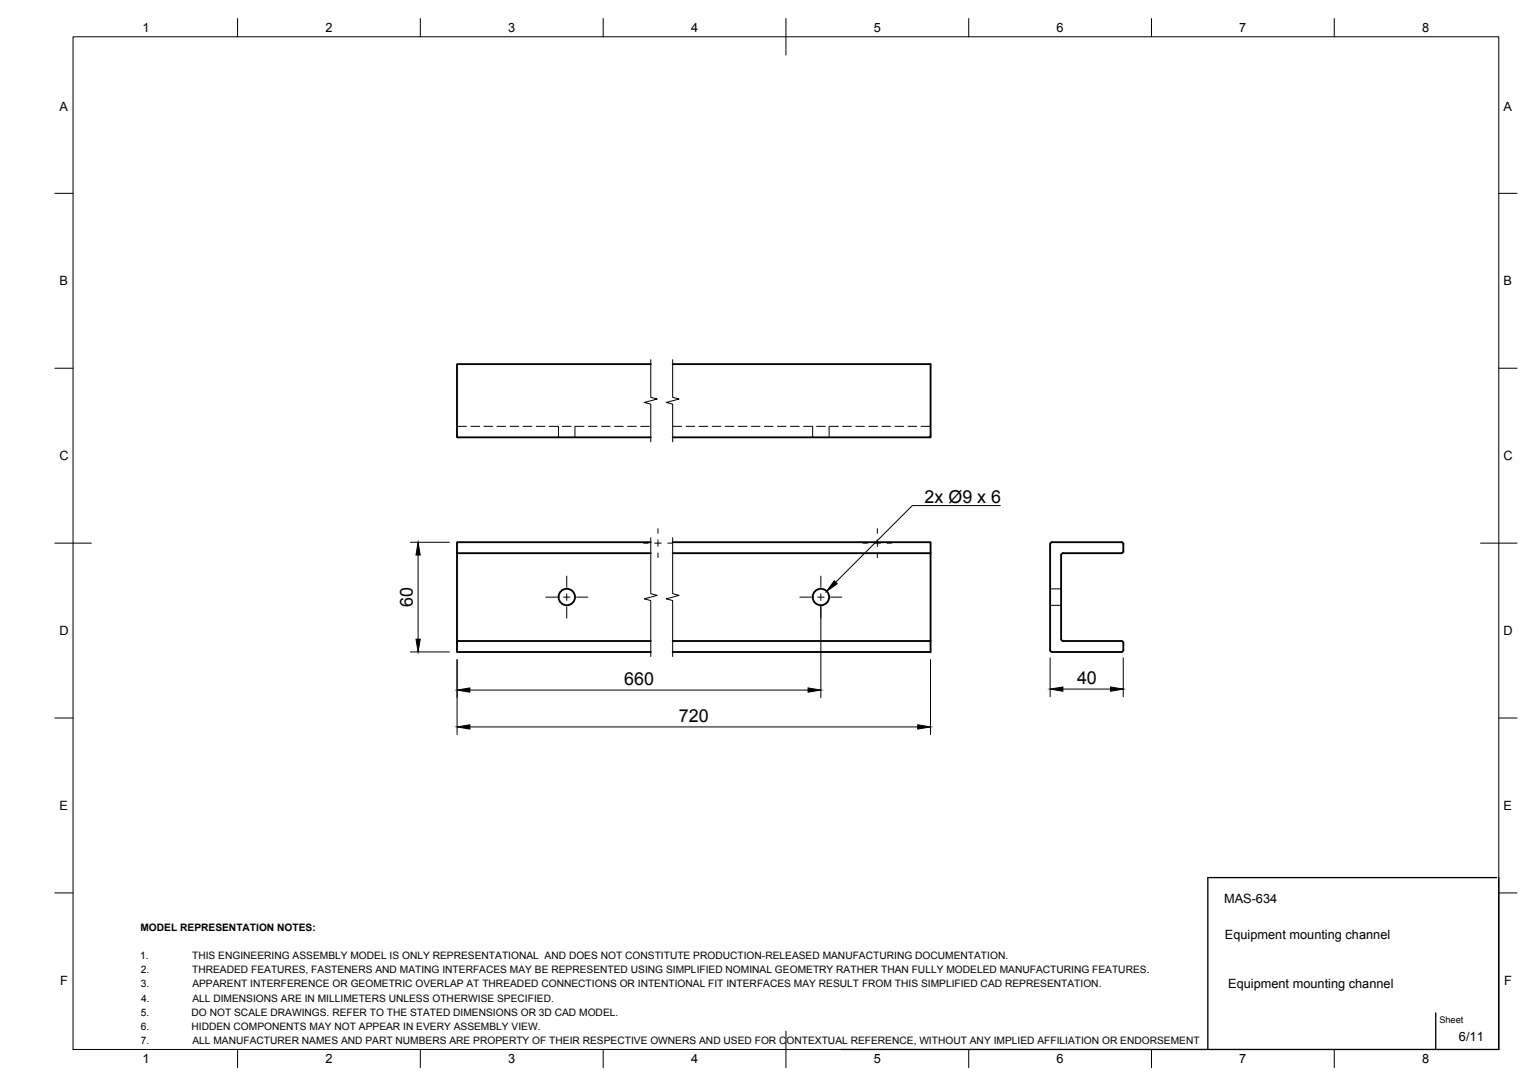
ISO-10303-21;
HEADER;
/* Generated by software containing ST-Developer
 * from STEP Tools, Inc. (www.steptools.com) 
 */

FILE_DESCRIPTION(
/* description */ ('Independent AHU equipment rack. Nominal800x600 frame on1000long40squa
re aluminum posts; two removable notched shelves; welded perimeter/cro
ss rails and rear gussets; two mounting channels; four isolation pads 
and anchor-ready feet. Imported native extrusion library retained and 
cut-length parameters customized per family. Shelf hardware uses model
ed M6 rivet nuts and screws. Weld design, floor anchors and load ratin
g require engineering selection.'),
/* implementation_level */ '2;1');

FILE_NAME(
/* name */ 'Equipment mounting channel.step',
/* time_stamp */ '2026-11-07T19:04:45-08:00',
/* author */ (''),
/* organization */ (''),
/* preprocessor_version */ 'ST-DEVELOPER v20.2',
/* originating_system */ 'Autodesk Translation Framework v15.17.0.0',
/* authorisation */ '');

FILE_SCHEMA (('AUTOMOTIVE_DESIGN { 1 0 10303 214 3 1 1 }'));
ENDSEC;

DATA;
#10=MECHANICAL_DESIGN_GEOMETRIC_PRESENTATION_REPRESENTATION('',(#338),#9777);
#316=SHAPE_REPRESENTATION_RELATIONSHIP('SRR','None',#9860,#327);
#327=ADVANCED_BREP_SHAPE_REPRESENTATION('',(#349),#9769);
#338=STYLED_ITEM('',(#9923),#349);
#349=MANIFOLD_SOLID_BREP('Aluminum channel profile',#3843);
#367=FACE_BOUND('',#771,.T.);
#368=FACE_BOUND('',#772,.T.);
#369=FACE_BOUND('',#779,.T.);
#370=FACE_BOUND('',#780,.T.);
#440=PLANE('',#4095);
#441=PLANE('',#4103);
#442=PLANE('',#4108);
#443=PLANE('',#4113);
#444=PLANE('',#4116);
#445=PLANE('',#4121);
#446=PLANE('',#4122);
#447=PLANE('',#4123);
#448=PLANE('',#4124);
#449=PLANE('',#4125);
#558=FACE_OUTER_BOUND('',#766,.T.);
#559=FACE_OUTER_BOUND('',#767,.T.);
#560=FACE_OUTER_BOUND('',#768,.T.);
#561=FACE_OUTER_BOUND('',#769,.T.);
#562=FACE_OUTER_BOUND('',#770,.T.);
#563=FACE_OUTER_BOUND('',#773,.T.);
#564=FACE_OUTER_BOUND('',#774,.T.);
#565=FACE_OUTER_BOUND('',#775,.T.);
#566=FACE_OUTER_BOUND('',#776,.T.);
#567=FACE_OUTER_BOUND('',#777,.T.);
#568=FACE_OUTER_BOUND('',#778,.T.);
#569=FACE_OUTER_BOUND('',#781,.T.);
#570=FACE_OUTER_BOUND('',#782,.T.);
#571=FACE_OUTER_BOUND('',#783,.T.);
#572=FACE_OUTER_BOUND('',#784,.T.);
#573=FACE_OUTER_BOUND('',#785,.T.);
#574=FACE_OUTER_BOUND('',#786,.T.);
#575=FACE_OUTER_BOUND('',#787,.T.);
#576=FACE_OUTER_BOUND('',#788,.T.);
#577=FACE_OUTER_BOUND('',#789,.T.);
#766=EDGE_LOOP('',(#2815,#2816,#2817,#2818));
#767=EDGE_LOOP('',(#2819,#2820,#2821,#2822));
#768=EDGE_LOOP('',(#2823,#2824,#2825,#2826));
#769=EDGE_LOOP('',(#2827,#2828,#2829,#2830,#2831,#2832,#2833,#2834,#2835,
#2836,#2837,#2838,#2839,#2840,#2841,#2842));
#770=EDGE_LOOP('',(#2843,#2844,#2845,#2846));
#771=EDGE_LOOP('',(#2847));
#772=EDGE_LOOP('',(#2848));
#773=EDGE_LOOP('',(#2849,#2850,#2851,#2852));
#774=EDGE_LOOP('',(#2853,#2854,#2855,#2856));
#775=EDGE_LOOP('',(#2857,#2858,#2859,#2860));
#776=EDGE_LOOP('',(#2861,#2862,#2863,#2864));
#777=EDGE_LOOP('',(#2865,#2866,#2867,#2868));
#778=EDGE_LOOP('',(#2869,#2870,#2871,#2872));
#779=EDGE_LOOP('',(#2873));
#780=EDGE_LOOP('',(#2874));
#781=EDGE_LOOP('',(#2875,#2876,#2877,#2878));
#782=EDGE_LOOP('',(#2879,#2880,#2881,#2882));
#783=EDGE_LOOP('',(#2883,#2884,#2885,#2886));
#784=EDGE_LOOP('',(#2887,#2888,#2889,#2890));
#785=EDGE_LOOP('',(#2891,#2892,#2893,#2894));
#786=EDGE_LOOP('',(#2895,#2896,#2897,#2898));
#787=EDGE_LOOP('',(#2899,#2900,#2901,#2902));
#788=EDGE_LOOP('',(#2903,#2904,#2905,#2906));
#789=EDGE_LOOP('',(#2907,#2908,#2909,#2910,#2911,#2912,#2913,#2914,#2915,
#2916,#2917,#2918,#2919,#2920,#2921,#2922));
#1049=LINE('',#5718,#1342);
#1050=LINE('',#5724,#1343);
#1051=LINE('',#5731,#1344);
#1052=LINE('',#5734,#1345);
#1053=LINE('',#5737,#1346);
#1054=LINE('',#5741,#1347);
#1055=LINE('',#5745,#1348);
#1056=LINE('',#5749,#1349);
#1057=LINE('',#5753,#1350);
#1058=LINE('',#5757,#1351);
#1059=LINE('',#5761,#1352);
#1060=LINE('',#5764,#1353);
#1061=LINE('',#5767,#1354);
#1062=LINE('',#5768,#1355);
#1063=LINE('',#5772,#1356);
#1064=LINE('',#5775,#1357);
#1065=LINE('',#5778,#1358);
#1066=LINE('',#5781,#1359);
#1067=LINE('',#5782,#1360);
#1068=LINE('',#5786,#1361);
#1069=LINE('',#5791,#1362);
#1070=LINE('',#5792,#1363);
#1071=LINE('',#5795,#1364);
#1072=LINE('',#5796,#1365);
#1073=LINE('',#5800,#1366);
#1074=LINE('',#5803,#1367);
#1075=LINE('',#5804,#1368);
#1076=LINE('',#5808,#1369);
#1077=LINE('',#5811,#1370);
#1078=LINE('',#5814,#1371);
#1079=LINE('',#5816,#1372);
#1080=LINE('',#5818,#1373);
#1081=LINE('',#5820,#1374);
#1082=LINE('',#5822,#1375);
#1342=VECTOR('',#4680,4.5);
#1343=VECTOR('',#4687,4.5);
#1344=VECTOR('',#4694,10.);
#1345=VECTOR('',#4697,10.);
#1346=VECTOR('',#4700,10.);
#1347=VECTOR('',#4703,10.);
#1348=VECTOR('',#4706,10.);
#1349=VECTOR('',#4709,10.);
#1350=VECTOR('',#4712,10.);
#1351=VECTOR('',#4715,10.);
#1352=VECTOR('',#4718,10.);
#1353=VECTOR('',#4721,10.);
#1354=VECTOR('',#4724,10.);
#1355=VECTOR('',#4725,10.);
#1356=VECTOR('',#4730,10.);
#1357=VECTOR('',#4733,10.);
#1358=VECTOR('',#4736,10.);
#1359=VECTOR('',#4739,10.);
#1360=VECTOR('',#4740,10.);
#1361=VECTOR('',#4745,10.);
#1362=VECTOR('',#4750,10.);
#1363=VECTOR('',#4751,10.);
#1364=VECTOR('',#4754,10.);
#1365=VECTOR('',#4755,10.);
#1366=VECTOR('',#4760,10.);
#1367=VECTOR('',#4763,10.);
#1368=VECTOR('',#4764,10.);
#1369=VECTOR('',#4769,10.);
#1370=VECTOR('',#4772,10.);
#1371=VECTOR('',#4775,10.);
#1372=VECTOR('',#4778,10.);
#1373=VECTOR('',#4781,10.);
#1374=VECTOR('',#4784,10.);
#1375=VECTOR('',#4787,10.);
#1589=CIRCLE('',#4087,4.5);
#1590=CIRCLE('',#4088,4.5);
#1591=CIRCLE('',#4090,4.5);
#1592=CIRCLE('',#4091,4.5);
#1593=CIRCLE('',#4093,1.);
#1594=CIRCLE('',#4094,1.);
#1595=CIRCLE('',#4096,1.);
#1596=CIRCLE('',#4097,1.);
#1597=CIRCLE('',#4098,1.);
#1598=CIRCLE('',#4099,1.);
#1599=CIRCLE('',#4100,1.);
#1600=CIRCLE('',#4101,1.);
#1601=CIRCLE('',#4102,1.);
#1602=CIRCLE('',#4105,1.);
#1603=CIRCLE('',#4107,1.);
#1604=CIRCLE('',#4110,1.);
#1605=CIRCLE('',#4112,1.);
#1606=CIRCLE('',#4115,1.);
#1607=CIRCLE('',#4118,1.);
#1608=CIRCLE('',#4120,1.);
#1760=VERTEX_POINT('',#5715);
#1761=VERTEX_POINT('',#5717);
#1762=VERTEX_POINT('',#5721);
#1763=VERTEX_POINT('',#5723);
#1764=VERTEX_POINT('',#5727);
#1765=VERTEX_POINT('',#5728);
#1766=VERTEX_POINT('',#5730);
#1767=VERTEX_POINT('',#5732);
#1768=VERTEX_POINT('',#5736);
#1769=VERTEX_POINT('',#5738);
#1770=VERTEX_POINT('',#5740);
#1771=VERTEX_POINT('',#5742);
#1772=VERTEX_POINT('',#5744);
#1773=VERTEX_POINT('',#5746);
#1774=VERTEX_POINT('',#5748);
#1775=VERTEX_POINT('',#5750);
#1776=VERTEX_POINT('',#5752);
#1777=VERTEX_POINT('',#5754);
#1778=VERTEX_POINT('',#5756);
#1779=VERTEX_POINT('',#5758);
#1780=VERTEX_POINT('',#5760);
#1781=VERTEX_POINT('',#5762);
#1782=VERTEX_POINT('',#5766);
#1783=VERTEX_POINT('',#5770);
#1784=VERTEX_POINT('',#5774);
#1785=VERTEX_POINT('',#5776);
#1786=VERTEX_POINT('',#5780);
#1787=VERTEX_POINT('',#5784);
#1788=VERTEX_POINT('',#5788);
#1789=VERTEX_POINT('',#5789);
#1790=VERTEX_POINT('',#5794);
#1791=VERTEX_POINT('',#5798);
#1792=VERTEX_POINT('',#5802);
#1793=VERTEX_POINT('',#5806);
#1794=VERTEX_POINT('',#5810);
#1795=VERTEX_POINT('',#5812);
#2152=EDGE_CURVE('',#1760,#1760,#1589,.T.);
#2153=EDGE_CURVE('',#1760,#1761,#1049,.T.);
#2154=EDGE_CURVE('',#1761,#1761,#1590,.T.);
#2155=EDGE_CURVE('',#1762,#1762,#1591,.T.);
#2156=EDGE_CURVE('',#1762,#1763,#1050,.T.);
#2157=EDGE_CURVE('',#1763,#1763,#1592,.T.);
#2158=EDGE_CURVE('',#1764,#1765,#1593,.T.);
#2159=EDGE_CURVE('',#1765,#1766,#1051,.T.);
#2160=EDGE_CURVE('',#1766,#1767,#1594,.T.);
#2161=EDGE_CURVE('',#1767,#1764,#1052,.T.);
#2162=EDGE_CURVE('',#1764,#1768,#1053,.T.);
#2163=EDGE_CURVE('',#1769,#1768,#1595,.T.);
#2164=EDGE_CURVE('',#1769,#1770,#1054,.T.);
#2165=EDGE_CURVE('',#1771,#1770,#1596,.T.);
#2166=EDGE_CURVE('',#1771,#1772,#1055,.T.);
#2167=EDGE_CURVE('',#1773,#1772,#1597,.T.);
#2168=EDGE_CURVE('',#1773,#1774,#1056,.T.);
#2169=EDGE_CURVE('',#1775,#1774,#1598,.T.);
#2170=EDGE_CURVE('',#1775,#1776,#1057,.T.);
#2171=EDGE_CURVE('',#1777,#1776,#1599,.T.);
#2172=EDGE_CURVE('',#1777,#1778,#1058,.T.);
#2173=EDGE_CURVE('',#1779,#1778,#1600,.T.);
#2174=EDGE_CURVE('',#1779,#1780,#1059,.T.);
#2175=EDGE_CURVE('',#1781,#1780,#1601,.T.);
#2176=EDGE_CURVE('',#1781,#1765,#1060,.T.);
#2177=EDGE_CURVE('',#1767,#1782,#1061,.T.);
#2178=EDGE_CURVE('',#1768,#1782,#1062,.T.);
#2179=EDGE_CURVE('',#1782,#1783,#1602,.T.);
#2180=EDGE_CURVE('',#1783,#1769,#1063,.T.);
#2181=EDGE_CURVE('',#1770,#1784,#1064,.T.);
#2182=EDGE_CURVE('',#1784,#1785,#1603,.T.);
#2183=EDGE_CURVE('',#1785,#1771,#1065,.T.);
#2184=EDGE_CURVE('',#1785,#1786,#1066,.T.);
#2185=EDGE_CURVE('',#1772,#1786,#1067,.T.);
#2186=EDGE_CURVE('',#1786,#1787,#1604,.T.);
#2187=EDGE_CURVE('',#1787,#1773,#1068,.T.);
#2188=EDGE_CURVE('',#1788,#1789,#1605,.T.);
#2189=EDGE_CURVE('',#1789,#1775,#1069,.T.);
#2190=EDGE_CURVE('',#1774,#1788,#1070,.T.);
#2191=EDGE_CURVE('',#1789,#1790,#1071,.T.);
#2192=EDGE_CURVE('',#1776,#1790,#1072,.T.);
#2193=EDGE_CURVE('',#1790,#1791,#1606,.T.);
#2194=EDGE_CURVE('',#1791,#1777,#1073,.T.);
#2195=EDGE_CURVE('',#1791,#1792,#1074,.T.);
#2196=EDGE_CURVE('',#1778,#1792,#1075,.T.);
#2197=EDGE_CURVE('',#1792,#1793,#1607,.T.);
#2198=EDGE_CURVE('',#1793,#1779,#1076,.T.);
#2199=EDGE_CURVE('',#1780,#1794,#1077,.T.);
#2200=EDGE_CURVE('',#1794,#1795,#1608,.T.);
#2201=EDGE_CURVE('',#1795,#1781,#1078,.T.);
#2202=EDGE_CURVE('',#1795,#1766,#1079,.T.);
#2203=EDGE_CURVE('',#1793,#1794,#1080,.T.);
#2204=EDGE_CURVE('',#1787,#1788,#1081,.T.);
#2205=EDGE_CURVE('',#1783,#1784,#1082,.T.);
#2815=ORIENTED_EDGE('',*,*,#2152,.F.);
#2816=ORIENTED_EDGE('',*,*,#2153,.T.);
#2817=ORIENTED_EDGE('',*,*,#2154,.F.);
#2818=ORIENTED_EDGE('',*,*,#2153,.F.);
#2819=ORIENTED_EDGE('',*,*,#2155,.F.);
#2820=ORIENTED_EDGE('',*,*,#2156,.T.);
#2821=ORIENTED_EDGE('',*,*,#2157,.F.);
#2822=ORIENTED_EDGE('',*,*,#2156,.F.);
#2823=ORIENTED_EDGE('',*,*,#2158,.T.);
#2824=ORIENTED_EDGE('',*,*,#2159,.T.);
#2825=ORIENTED_EDGE('',*,*,#2160,.T.);
#2826=ORIENTED_EDGE('',*,*,#2161,.T.);
#2827=ORIENTED_EDGE('',*,*,#2158,.F.);
#2828=ORIENTED_EDGE('',*,*,#2162,.T.);
#2829=ORIENTED_EDGE('',*,*,#2163,.F.);
#2830=ORIENTED_EDGE('',*,*,#2164,.T.);
#2831=ORIENTED_EDGE('',*,*,#2165,.F.);
#2832=ORIENTED_EDGE('',*,*,#2166,.T.);
#2833=ORIENTED_EDGE('',*,*,#2167,.F.);
#2834=ORIENTED_EDGE('',*,*,#2168,.T.);
#2835=ORIENTED_EDGE('',*,*,#2169,.F.);
#2836=ORIENTED_EDGE('',*,*,#2170,.T.);
#2837=ORIENTED_EDGE('',*,*,#2171,.F.);
#2838=ORIENTED_EDGE('',*,*,#2172,.T.);
#2839=ORIENTED_EDGE('',*,*,#2173,.F.);
#2840=ORIENTED_EDGE('',*,*,#2174,.T.);
#2841=ORIENTED_EDGE('',*,*,#2175,.F.);
#2842=ORIENTED_EDGE('',*,*,#2176,.T.);
#2843=ORIENTED_EDGE('',*,*,#2161,.F.);
#2844=ORIENTED_EDGE('',*,*,#2177,.T.);
#2845=ORIENTED_EDGE('',*,*,#2178,.F.);
#2846=ORIENTED_EDGE('',*,*,#2162,.F.);
#2847=ORIENTED_EDGE('',*,*,#2154,.T.);
#2848=ORIENTED_EDGE('',*,*,#2157,.T.);
#2849=ORIENTED_EDGE('',*,*,#2163,.T.);
#2850=ORIENTED_EDGE('',*,*,#2178,.T.);
#2851=ORIENTED_EDGE('',*,*,#2179,.T.);
#2852=ORIENTED_EDGE('',*,*,#2180,.T.);
#2853=ORIENTED_EDGE('',*,*,#2165,.T.);
#2854=ORIENTED_EDGE('',*,*,#2181,.T.);
#2855=ORIENTED_EDGE('',*,*,#2182,.T.);
#2856=ORIENTED_EDGE('',*,*,#2183,.T.);
#2857=ORIENTED_EDGE('',*,*,#2183,.F.);
#2858=ORIENTED_EDGE('',*,*,#2184,.T.);
#2859=ORIENTED_EDGE('',*,*,#2185,.F.);
#2860=ORIENTED_EDGE('',*,*,#2166,.F.);
#2861=ORIENTED_EDGE('',*,*,#2167,.T.);
#2862=ORIENTED_EDGE('',*,*,#2185,.T.);
#2863=ORIENTED_EDGE('',*,*,#2186,.T.);
#2864=ORIENTED_EDGE('',*,*,#2187,.T.);
#2865=ORIENTED_EDGE('',*,*,#2188,.T.);
#2866=ORIENTED_EDGE('',*,*,#2189,.T.);
#2867=ORIENTED_EDGE('',*,*,#2169,.T.);
#2868=ORIENTED_EDGE('',*,*,#2190,.T.);
#2869=ORIENTED_EDGE('',*,*,#2189,.F.);
#2870=ORIENTED_EDGE('',*,*,#2191,.T.);
#2871=ORIENTED_EDGE('',*,*,#2192,.F.);
#2872=ORIENTED_EDGE('',*,*,#2170,.F.);
#2873=ORIENTED_EDGE('',*,*,#2152,.T.);
#2874=ORIENTED_EDGE('',*,*,#2155,.T.);
#2875=ORIENTED_EDGE('',*,*,#2193,.T.);
#2876=ORIENTED_EDGE('',*,*,#2194,.T.);
#2877=ORIENTED_EDGE('',*,*,#2171,.T.);
#2878=ORIENTED_EDGE('',*,*,#2192,.T.);
#2879=ORIENTED_EDGE('',*,*,#2194,.F.);
#2880=ORIENTED_EDGE('',*,*,#2195,.T.);
#2881=ORIENTED_EDGE('',*,*,#2196,.F.);
#2882=ORIENTED_EDGE('',*,*,#2172,.F.);
#2883=ORIENTED_EDGE('',*,*,#2173,.T.);
#2884=ORIENTED_EDGE('',*,*,#2196,.T.);
#2885=ORIENTED_EDGE('',*,*,#2197,.T.);
#2886=ORIENTED_EDGE('',*,*,#2198,.T.);
#2887=ORIENTED_EDGE('',*,*,#2175,.T.);
#2888=ORIENTED_EDGE('',*,*,#2199,.T.);
#2889=ORIENTED_EDGE('',*,*,#2200,.T.);
#2890=ORIENTED_EDGE('',*,*,#2201,.T.);
#2891=ORIENTED_EDGE('',*,*,#2159,.F.);
#2892=ORIENTED_EDGE('',*,*,#2176,.F.);
#2893=ORIENTED_EDGE('',*,*,#2201,.F.);
#2894=ORIENTED_EDGE('',*,*,#2202,.T.);
#2895=ORIENTED_EDGE('',*,*,#2198,.F.);
#2896=ORIENTED_EDGE('',*,*,#2203,.T.);
#2897=ORIENTED_EDGE('',*,*,#2199,.F.);
#2898=ORIENTED_EDGE('',*,*,#2174,.F.);
#2899=ORIENTED_EDGE('',*,*,#2187,.F.);
#2900=ORIENTED_EDGE('',*,*,#2204,.T.);
#2901=ORIENTED_EDGE('',*,*,#2190,.F.);
#2902=ORIENTED_EDGE('',*,*,#2168,.F.);
#2903=ORIENTED_EDGE('',*,*,#2180,.F.);
#2904=ORIENTED_EDGE('',*,*,#2205,.T.);
#2905=ORIENTED_EDGE('',*,*,#2181,.F.);
#2906=ORIENTED_EDGE('',*,*,#2164,.F.);
#2907=ORIENTED_EDGE('',*,*,#2160,.F.);
#2908=ORIENTED_EDGE('',*,*,#2202,.F.);
#2909=ORIENTED_EDGE('',*,*,#2200,.F.);
#2910=ORIENTED_EDGE('',*,*,#2203,.F.);
#2911=ORIENTED_EDGE('',*,*,#2197,.F.);
#2912=ORIENTED_EDGE('',*,*,#2195,.F.);
#2913=ORIENTED_EDGE('',*,*,#2193,.F.);
#2914=ORIENTED_EDGE('',*,*,#2191,.F.);
#2915=ORIENTED_EDGE('',*,*,#2188,.F.);
#2916=ORIENTED_EDGE('',*,*,#2204,.F.);
#2917=ORIENTED_EDGE('',*,*,#2186,.F.);
#2918=ORIENTED_EDGE('',*,*,#2184,.F.);
#2919=ORIENTED_EDGE('',*,*,#2182,.F.);
#2920=ORIENTED_EDGE('',*,*,#2205,.F.);
#2921=ORIENTED_EDGE('',*,*,#2179,.F.);
#2922=ORIENTED_EDGE('',*,*,#2177,.F.);
#3567=CYLINDRICAL_SURFACE('',#4086,4.5);
#3568=CYLINDRICAL_SURFACE('',#4089,4.5);
#3569=CYLINDRICAL_SURFACE('',#4092,1.);
#3570=CYLINDRICAL_SURFACE('',#4104,1.);
#3571=CYLINDRICAL_SURFACE('',#4106,1.);
#3572=CYLINDRICAL_SURFACE('',#4109,1.);
#3573=CYLINDRICAL_SURFACE('',#4111,1.);
#3574=CYLINDRICAL_SURFACE('',#4114,1.);
#3575=CYLINDRICAL_SURFACE('',#4117,1.);
#3576=CYLINDRICAL_SURFACE('',#4119,1.);
#3698=ADVANCED_FACE('',(#558),#3567,.F.);
#3699=ADVANCED_FACE('',(#559),#3568,.F.);
#3700=ADVANCED_FACE('',(#560),#3569,.T.);
#3701=ADVANCED_FACE('',(#561),#440,.T.);
#3702=ADVANCED_FACE('',(#562,#367,#368),#441,.T.);
#3703=ADVANCED_FACE('',(#563),#3570,.T.);
#3704=ADVANCED_FACE('',(#564),#3571,.T.);
#3705=ADVANCED_FACE('',(#565),#442,.T.);
#3706=ADVANCED_FACE('',(#566),#3572,.T.);
#3707=ADVANCED_FACE('',(#567),#3573,.F.);
#3708=ADVANCED_FACE('',(#568,#369,#370),#443,.T.);
#3709=ADVANCED_FACE('',(#569),#3574,.F.);
#3710=ADVANCED_FACE('',(#570),#444,.T.);
#3711=ADVANCED_FACE('',(#571),#3575,.T.);
#3712=ADVANCED_FACE('',(#572),#3576,.T.);
#3713=ADVANCED_FACE('',(#573),#445,.T.);
#3714=ADVANCED_FACE('',(#574),#446,.T.);
#3715=ADVANCED_FACE('',(#575),#447,.T.);
#3716=ADVANCED_FACE('',(#576),#448,.T.);
#3717=ADVANCED_FACE('',(#577),#449,.F.);
#3843=CLOSED_SHELL('',(#3698,#3699,#3700,#3701,#3702,#3703,#3704,#3705,
#3706,#3707,#3708,#3709,#3710,#3711,#3712,#3713,#3714,#3715,#3716,#3717));
#4085=AXIS2_PLACEMENT_3D('',#5713,#4674,#4675);
#4086=AXIS2_PLACEMENT_3D('',#5714,#4676,#4677);
#4087=AXIS2_PLACEMENT_3D('',#5716,#4678,#4679);
#4088=AXIS2_PLACEMENT_3D('',#5719,#4681,#4682);
#4089=AXIS2_PLACEMENT_3D('',#5720,#4683,#4684);
#4090=AXIS2_PLACEMENT_3D('',#5722,#4685,#4686);
#4091=AXIS2_PLACEMENT_3D('',#5725,#4688,#4689);
#4092=AXIS2_PLACEMENT_3D('',#5726,#4690,#4691);
#4093=AXIS2_PLACEMENT_3D('',#5729,#4692,#4693);
#4094=AXIS2_PLACEMENT_3D('',#5733,#4695,#4696);
#4095=AXIS2_PLACEMENT_3D('',#5735,#4698,#4699);
#4096=AXIS2_PLACEMENT_3D('',#5739,#4701,#4702);
#4097=AXIS2_PLACEMENT_3D('',#5743,#4704,#4705);
#4098=AXIS2_PLACEMENT_3D('',#5747,#4707,#4708);
#4099=AXIS2_PLACEMENT_3D('',#5751,#4710,#4711);
#4100=AXIS2_PLACEMENT_3D('',#5755,#4713,#4714);
#4101=AXIS2_PLACEMENT_3D('',#5759,#4716,#4717);
#4102=AXIS2_PLACEMENT_3D('',#5763,#4719,#4720);
#4103=AXIS2_PLACEMENT_3D('',#5765,#4722,#4723);
#4104=AXIS2_PLACEMENT_3D('',#5769,#4726,#4727);
#4105=AXIS2_PLACEMENT_3D('',#5771,#4728,#4729);
#4106=AXIS2_PLACEMENT_3D('',#5773,#4731,#4732);
#4107=AXIS2_PLACEMENT_3D('',#5777,#4734,#4735);
#4108=AXIS2_PLACEMENT_3D('',#5779,#4737,#4738);
#4109=AXIS2_PLACEMENT_3D('',#5783,#4741,#4742);
#4110=AXIS2_PLACEMENT_3D('',#5785,#4743,#4744);
#4111=AXIS2_PLACEMENT_3D('',#5787,#4746,#4747);
#4112=AXIS2_PLACEMENT_3D('',#5790,#4748,#4749);
#4113=AXIS2_PLACEMENT_3D('',#5793,#4752,#4753);
#4114=AXIS2_PLACEMENT_3D('',#5797,#4756,#4757);
#4115=AXIS2_PLACEMENT_3D('',#5799,#4758,#4759);
#4116=AXIS2_PLACEMENT_3D('',#5801,#4761,#4762);
#4117=AXIS2_PLACEMENT_3D('',#5805,#4765,#4766);
#4118=AXIS2_PLACEMENT_3D('',#5807,#4767,#4768);
#4119=AXIS2_PLACEMENT_3D('',#5809,#4770,#4771);
#4120=AXIS2_PLACEMENT_3D('',#5813,#4773,#4774);
#4121=AXIS2_PLACEMENT_3D('',#5815,#4776,#4777);
#4122=AXIS2_PLACEMENT_3D('',#5817,#4779,#4780);
#4123=AXIS2_PLACEMENT_3D('',#5819,#4782,#4783);
#4124=AXIS2_PLACEMENT_3D('',#5821,#4785,#4786);
#4125=AXIS2_PLACEMENT_3D('',#5823,#4788,#4789);
#4674=DIRECTION('axis',(0.,0.,1.));
#4675=DIRECTION('refdir',(1.,0.,0.));
#4676=DIRECTION('center_axis',(0.,-1.,0.));
#4677=DIRECTION('ref_axis',(0.,0.,1.));
#4678=DIRECTION('center_axis',(0.,-1.,0.));
#4679=DIRECTION('ref_axis',(0.,0.,1.));
#4680=DIRECTION('',(0.,-1.,0.));
#4681=DIRECTION('center_axis',(0.,1.,0.));
#4682=DIRECTION('ref_axis',(0.,0.,1.));
#4683=DIRECTION('center_axis',(0.,-1.,0.));
#4684=DIRECTION('ref_axis',(0.,0.,1.));
#4685=DIRECTION('center_axis',(0.,-1.,0.));
#4686=DIRECTION('ref_axis',(0.,0.,1.));
#4687=DIRECTION('',(0.,-1.,0.));
#4688=DIRECTION('center_axis',(0.,1.,0.));
#4689=DIRECTION('ref_axis',(0.,0.,1.));
#4690=DIRECTION('center_axis',(0.,0.,1.));
#4691=DIRECTION('ref_axis',(-0.707106781186547,-0.707106781186548,0.));
#4692=DIRECTION('center_axis',(0.,0.,-1.));
#4693=DIRECTION('ref_axis',(-0.707106781186547,-0.707106781186548,0.));
#4694=DIRECTION('',(0.,0.,-1.));
#4695=DIRECTION('center_axis',(0.,0.,1.));
#4696=DIRECTION('ref_axis',(-0.707106781186547,-0.707106781186548,0.));
#4697=DIRECTION('',(0.,0.,1.));
#4698=DIRECTION('center_axis',(0.,0.,1.));
#4699=DIRECTION('ref_axis',(1.,0.,0.));
#4700=DIRECTION('',(1.,0.,0.));
#4701=DIRECTION('center_axis',(0.,0.,-1.));
#4702=DIRECTION('ref_axis',(0.707106781186546,-0.707106781186549,0.));
#4703=DIRECTION('',(0.,1.,0.));
#4704=DIRECTION('center_axis',(0.,0.,-1.));
#4705=DIRECTION('ref_axis',(0.707106781186544,0.707106781186551,0.));
#4706=DIRECTION('',(-1.,0.,0.));
#4707=DIRECTION('center_axis',(0.,0.,-1.));
#4708=DIRECTION('ref_axis',(-0.707106781186548,0.707106781186548,0.));
#4709=DIRECTION('',(0.,-1.,0.));
#4710=DIRECTION('center_axis',(0.,0.,1.));
#4711=DIRECTION('ref_axis',(0.707106781186546,-0.707106781186549,0.));
#4712=DIRECTION('',(-1.,0.,0.));
#4713=DIRECTION('center_axis',(0.,0.,1.));
#4714=DIRECTION('ref_axis',(-0.707106781186546,-0.707106781186549,0.));
#4715=DIRECTION('',(0.,1.,0.));
#4716=DIRECTION('center_axis',(0.,0.,-1.));
#4717=DIRECTION('ref_axis',(0.707106781186546,0.707106781186549,0.));
#4718=DIRECTION('',(-1.,0.,0.));
#4719=DIRECTION('center_axis',(0.,0.,-1.));
#4720=DIRECTION('ref_axis',(-0.707106781186549,0.707106781186546,0.));
#4721=DIRECTION('',(0.,-1.,0.));
#4722=DIRECTION('center_axis',(0.,-1.,0.));
#4723=DIRECTION('ref_axis',(1.,0.,0.));
#4724=DIRECTION('',(1.,0.,0.));
#4725=DIRECTION('',(0.,0.,-1.));
#4726=DIRECTION('center_axis',(0.,0.,1.));
#4727=DIRECTION('ref_axis',(0.707106781186546,-0.707106781186549,0.));
#4728=DIRECTION('center_axis',(0.,0.,1.));
#4729=DIRECTION('ref_axis',(0.707106781186546,-0.707106781186549,0.));
#4730=DIRECTION('',(0.,0.,1.));
#4731=DIRECTION('center_axis',(0.,0.,1.));
#4732=DIRECTION('ref_axis',(0.707106781186544,0.707106781186551,0.));
#4733=DIRECTION('',(0.,0.,-1.));
#4734=DIRECTION('center_axis',(0.,0.,1.));
#4735=DIRECTION('ref_axis',(0.707106781186544,0.707106781186551,0.));
#4736=DIRECTION('',(0.,0.,1.));
#4737=DIRECTION('center_axis',(0.,1.,0.));
#4738=DIRECTION('ref_axis',(-1.,0.,0.));
#4739=DIRECTION('',(-1.,0.,0.));
#4740=DIRECTION('',(0.,0.,-1.));
#4741=DIRECTION('center_axis',(0.,0.,1.));
#4742=DIRECTION('ref_axis',(-0.707106781186548,0.707106781186548,0.));
#4743=DIRECTION('center_axis',(0.,0.,1.));
#4744=DIRECTION('ref_axis',(-0.707106781186548,0.707106781186548,0.));
#4745=DIRECTION('',(0.,0.,1.));
#4746=DIRECTION('center_axis',(0.,0.,1.));
#4747=DIRECTION('ref_axis',(0.707106781186546,-0.707106781186549,0.));
#4748=DIRECTION('center_axis',(0.,0.,-1.));
#4749=DIRECTION('ref_axis',(0.707106781186546,-0.707106781186549,0.));
#4750=DIRECTION('',(0.,0.,1.));
#4751=DIRECTION('',(0.,0.,-1.));
#4752=DIRECTION('center_axis',(0.,1.,0.));
#4753=DIRECTION('ref_axis',(-1.,0.,0.));
#4754=DIRECTION('',(-1.,0.,0.));
#4755=DIRECTION('',(0.,0.,-1.));
#4756=DIRECTION('center_axis',(0.,0.,1.));
#4757=DIRECTION('ref_axis',(-0.707106781186546,-0.707106781186549,0.));
#4758=DIRECTION('center_axis',(0.,0.,-1.));
#4759=DIRECTION('ref_axis',(-0.707106781186546,-0.707106781186549,0.));
#4760=DIRECTION('',(0.,0.,1.));
#4761=DIRECTION('center_axis',(1.,0.,0.));
#4762=DIRECTION('ref_axis',(0.,1.,0.));
#4763=DIRECTION('',(0.,1.,0.));
#4764=DIRECTION('',(0.,0.,-1.));
#4765=DIRECTION('center_axis',(0.,0.,1.));
#4766=DIRECTION('ref_axis',(0.707106781186546,0.707106781186549,0.));
#4767=DIRECTION('center_axis',(0.,0.,1.));
#4768=DIRECTION('ref_axis',(0.707106781186546,0.707106781186549,0.));
#4769=DIRECTION('',(0.,0.,1.));
#4770=DIRECTION('center_axis',(0.,0.,1.));
#4771=DIRECTION('ref_axis',(-0.707106781186549,0.707106781186546,0.));
#4772=DIRECTION('',(0.,0.,-1.));
#4773=DIRECTION('center_axis',(0.,0.,1.));
#4774=DIRECTION('ref_axis',(-0.707106781186549,0.707106781186546,0.));
#4775=DIRECTION('',(0.,0.,1.));
#4776=DIRECTION('center_axis',(-1.,0.,0.));
#4777=DIRECTION('ref_axis',(0.,-1.,0.));
#4778=DIRECTION('',(0.,-1.,0.));
#4779=DIRECTION('center_axis',(0.,1.,0.));
#4780=DIRECTION('ref_axis',(-1.,0.,0.));
#4781=DIRECTION('',(-1.,0.,0.));
#4782=DIRECTION('center_axis',(-1.,0.,0.));
#4783=DIRECTION('ref_axis',(0.,-1.,0.));
#4784=DIRECTION('',(0.,-1.,0.));
#4785=DIRECTION('center_axis',(1.,0.,0.));
#4786=DIRECTION('ref_axis',(0.,1.,0.));
#4787=DIRECTION('',(0.,1.,0.));
#4788=DIRECTION('center_axis',(0.,0.,1.));
#4789=DIRECTION('ref_axis',(1.,0.,0.));
#5713=CARTESIAN_POINT('',(0.,0.,0.));
#5714=CARTESIAN_POINT('Origin',(30.,3.,60.));
#5715=CARTESIAN_POINT('',(30.,6.,55.5));
#5716=CARTESIAN_POINT('Origin',(30.,6.,60.));
#5717=CARTESIAN_POINT('',(30.,0.,55.5));
#5718=CARTESIAN_POINT('',(30.,3.,55.5));
#5719=CARTESIAN_POINT('Origin',(30.,0.,60.));
#5720=CARTESIAN_POINT('Origin',(30.,3.,660.));
#5721=CARTESIAN_POINT('',(30.,6.,655.5));
#5722=CARTESIAN_POINT('Origin',(30.,6.,660.));
#5723=CARTESIAN_POINT('',(30.,0.,655.5));
#5724=CARTESIAN_POINT('',(30.,3.,655.5));
#5725=CARTESIAN_POINT('Origin',(30.,0.,660.));
#5726=CARTESIAN_POINT('Origin',(1.,1.,0.));
#5727=CARTESIAN_POINT('',(1.,0.,720.));
#5728=CARTESIAN_POINT('',(0.,1.,720.));
#5729=CARTESIAN_POINT('Origin',(1.,1.,720.));
#5730=CARTESIAN_POINT('',(0.,1.,0.));
#5731=CARTESIAN_POINT('',(0.,1.,0.));
#5732=CARTESIAN_POINT('',(1.,0.,0.));
#5733=CARTESIAN_POINT('Origin',(1.,1.,0.));
#5734=CARTESIAN_POINT('',(1.,0.,0.));
#5735=CARTESIAN_POINT('Origin',(30.,20.,720.));
#5736=CARTESIAN_POINT('',(59.,0.,720.));
#5737=CARTESIAN_POINT('',(0.,0.,720.));
#5738=CARTESIAN_POINT('',(60.,1.,720.));
#5739=CARTESIAN_POINT('Origin',(59.,1.,720.));
#5740=CARTESIAN_POINT('',(60.,39.,720.));
#5741=CARTESIAN_POINT('',(60.,0.,720.));
#5742=CARTESIAN_POINT('',(59.,40.,720.));
#5743=CARTESIAN_POINT('Origin',(59.,39.,720.));
#5744=CARTESIAN_POINT('',(55.,40.,720.));
#5745=CARTESIAN_POINT('',(60.,40.,720.));
#5746=CARTESIAN_POINT('',(54.,39.,720.));
#5747=CARTESIAN_POINT('Origin',(55.,39.,720.));
#5748=CARTESIAN_POINT('',(54.,7.,720.));
#5749=CARTESIAN_POINT('',(54.,40.,720.));
#5750=CARTESIAN_POINT('',(53.,6.,720.));
#5751=CARTESIAN_POINT('Origin',(53.,7.,720.));
#5752=CARTESIAN_POINT('',(6.99999999999999,6.,720.));
#5753=CARTESIAN_POINT('',(54.,6.,720.));
#5754=CARTESIAN_POINT('',(6.,7.,720.));
#5755=CARTESIAN_POINT('Origin',(7.,7.,720.));
#5756=CARTESIAN_POINT('',(6.,39.,720.));
#5757=CARTESIAN_POINT('',(6.,6.,720.));
#5758=CARTESIAN_POINT('',(5.,40.,720.));
#5759=CARTESIAN_POINT('Origin',(5.,39.,720.));
#5760=CARTESIAN_POINT('',(1.,40.,720.));
#5761=CARTESIAN_POINT('',(6.,40.,720.));
#5762=CARTESIAN_POINT('',(0.,39.,720.));
#5763=CARTESIAN_POINT('Origin',(1.,39.,720.));
#5764=CARTESIAN_POINT('',(0.,40.,720.));
#5765=CARTESIAN_POINT('Origin',(0.,0.,0.));
#5766=CARTESIAN_POINT('',(59.,0.,0.));
#5767=CARTESIAN_POINT('',(0.,0.,0.));
#5768=CARTESIAN_POINT('',(59.,0.,0.));
#5769=CARTESIAN_POINT('Origin',(59.,1.,0.));
#5770=CARTESIAN_POINT('',(60.,1.,0.));
#5771=CARTESIAN_POINT('Origin',(59.,1.,0.));
#5772=CARTESIAN_POINT('',(60.,1.,0.));
#5773=CARTESIAN_POINT('Origin',(59.,39.,0.));
#5774=CARTESIAN_POINT('',(60.,39.,0.));
#5775=CARTESIAN_POINT('',(60.,39.,0.));
#5776=CARTESIAN_POINT('',(59.,40.,0.));
#5777=CARTESIAN_POINT('Origin',(59.,39.,0.));
#5778=CARTESIAN_POINT('',(59.,40.,0.));
#5779=CARTESIAN_POINT('Origin',(60.,40.,0.));
#5780=CARTESIAN_POINT('',(55.,40.,0.));
#5781=CARTESIAN_POINT('',(60.,40.,0.));
#5782=CARTESIAN_POINT('',(55.,40.,0.));
#5783=CARTESIAN_POINT('Origin',(55.,39.,0.));
#5784=CARTESIAN_POINT('',(54.,39.,0.));
#5785=CARTESIAN_POINT('Origin',(55.,39.,0.));
#5786=CARTESIAN_POINT('',(54.,39.,0.));
#5787=CARTESIAN_POINT('Origin',(53.,7.,0.));
#5788=CARTESIAN_POINT('',(54.,7.,0.));
#5789=CARTESIAN_POINT('',(53.,6.,0.));
#5790=CARTESIAN_POINT('Origin',(53.,7.,0.));
#5791=CARTESIAN_POINT('',(53.,6.,0.));
#5792=CARTESIAN_POINT('',(54.,7.,0.));
#5793=CARTESIAN_POINT('Origin',(54.,6.,0.));
#5794=CARTESIAN_POINT('',(6.99999999999999,6.,0.));
#5795=CARTESIAN_POINT('',(54.,6.,0.));
#5796=CARTESIAN_POINT('',(7.,6.,0.));
#5797=CARTESIAN_POINT('Origin',(7.,7.,0.));
#5798=CARTESIAN_POINT('',(6.,7.,0.));
#5799=CARTESIAN_POINT('Origin',(7.,7.,0.));
#5800=CARTESIAN_POINT('',(6.,7.,0.));
#5801=CARTESIAN_POINT('Origin',(6.,6.,0.));
#5802=CARTESIAN_POINT('',(6.,39.,0.));
#5803=CARTESIAN_POINT('',(6.,6.,0.));
#5804=CARTESIAN_POINT('',(6.,39.,0.));
#5805=CARTESIAN_POINT('Origin',(5.,39.,0.));
#5806=CARTESIAN_POINT('',(5.,40.,0.));
#5807=CARTESIAN_POINT('Origin',(5.,39.,0.));
#5808=CARTESIAN_POINT('',(5.,40.,0.));
#5809=CARTESIAN_POINT('Origin',(1.,39.,0.));
#5810=CARTESIAN_POINT('',(1.,40.,0.));
#5811=CARTESIAN_POINT('',(1.,40.,0.));
#5812=CARTESIAN_POINT('',(0.,39.,0.));
#5813=CARTESIAN_POINT('Origin',(1.,39.,0.));
#5814=CARTESIAN_POINT('',(0.,39.,0.));
#5815=CARTESIAN_POINT('Origin',(0.,40.,0.));
#5816=CARTESIAN_POINT('',(0.,40.,0.));
#5817=CARTESIAN_POINT('Origin',(6.,40.,0.));
#5818=CARTESIAN_POINT('',(6.,40.,0.));
#5819=CARTESIAN_POINT('Origin',(54.,40.,0.));
#5820=CARTESIAN_POINT('',(54.,40.,0.));
#5821=CARTESIAN_POINT('Origin',(60.,0.,0.));
#5822=CARTESIAN_POINT('',(60.,0.,0.));
#5823=CARTESIAN_POINT('Origin',(30.,20.,0.));
#9756=UNCERTAINTY_MEASURE_WITH_UNIT(LENGTH_MEASURE(0.01),#9778,
'DISTANCE_ACCURACY_VALUE',
'Maximum model space distance between geometric entities at asserted c
onnectivities');
#9764=UNCERTAINTY_MEASURE_WITH_UNIT(LENGTH_MEASURE(0.01),#9778,
'DISTANCE_ACCURACY_VALUE',
'Maximum model space distance between geometric entities at asserted c
onnectivities');
#9769=(
GEOMETRIC_REPRESENTATION_CONTEXT(3)
GLOBAL_UNCERTAINTY_ASSIGNED_CONTEXT((#9756))
GLOBAL_UNIT_ASSIGNED_CONTEXT((#9778,#9780,#9781))
REPRESENTATION_CONTEXT('','3D')
);
#9777=(
GEOMETRIC_REPRESENTATION_CONTEXT(3)
GLOBAL_UNCERTAINTY_ASSIGNED_CONTEXT((#9764))
GLOBAL_UNIT_ASSIGNED_CONTEXT((#9778,#9780,#9781))
REPRESENTATION_CONTEXT('','3D')
);
#9778=(
LENGTH_UNIT()
NAMED_UNIT(*)
SI_UNIT(.MILLI.,.METRE.)
);
#9780=(
NAMED_UNIT(*)
PLANE_ANGLE_UNIT()
SI_UNIT($,.RADIAN.)
);
#9781=(
NAMED_UNIT(*)
SI_UNIT($,.STERADIAN.)
SOLID_ANGLE_UNIT()
);
#9786=SHAPE_DEFINITION_REPRESENTATION(#9798,#9860);
#9798=PRODUCT_DEFINITION_SHAPE('',$,#9873);
#9860=SHAPE_REPRESENTATION('',(#4085),#9769);
#9868=PRODUCT_DEFINITION_CONTEXT('part definition',#9906,'design');
#9873=PRODUCT_DEFINITION('Equipment mounting channel',
'Equipment mounting channel',#9885,#9868);
#9885=PRODUCT_DEFINITION_FORMATION('',$,#9912);
#9906=APPLICATION_CONTEXT(
'Core Data for Automotive Mechanical Design Process');
#9907=PRODUCT_CONTEXT('part definition',#9906,'mechanical');
#9912=PRODUCT('Equipment mounting channel','Equipment mounting channel',

'Independent aluminum extrusion section. Whole-mm nominal die dimensio
ns; parametric saw-cut length. Select structural loading, tolerances a
nd finish for the assembly application.',(#9907));
#9923=PRESENTATION_STYLE_ASSIGNMENT((#9934));
#9934=SURFACE_STYLE_USAGE(.BOTH.,#9945);
#9945=SURFACE_SIDE_STYLE('',(#9956));
#9956=SURFACE_STYLE_FILL_AREA(#9967);
#9967=FILL_AREA_STYLE('Sky blue',(#9978));
#9978=FILL_AREA_STYLE_COLOUR('Sky blue',#9989);
#9989=COLOUR_RGB('Sky blue',0.317647058823529,0.686274509803922,0.890196078431372);
ENDSEC;
END-ISO-10303-21;
